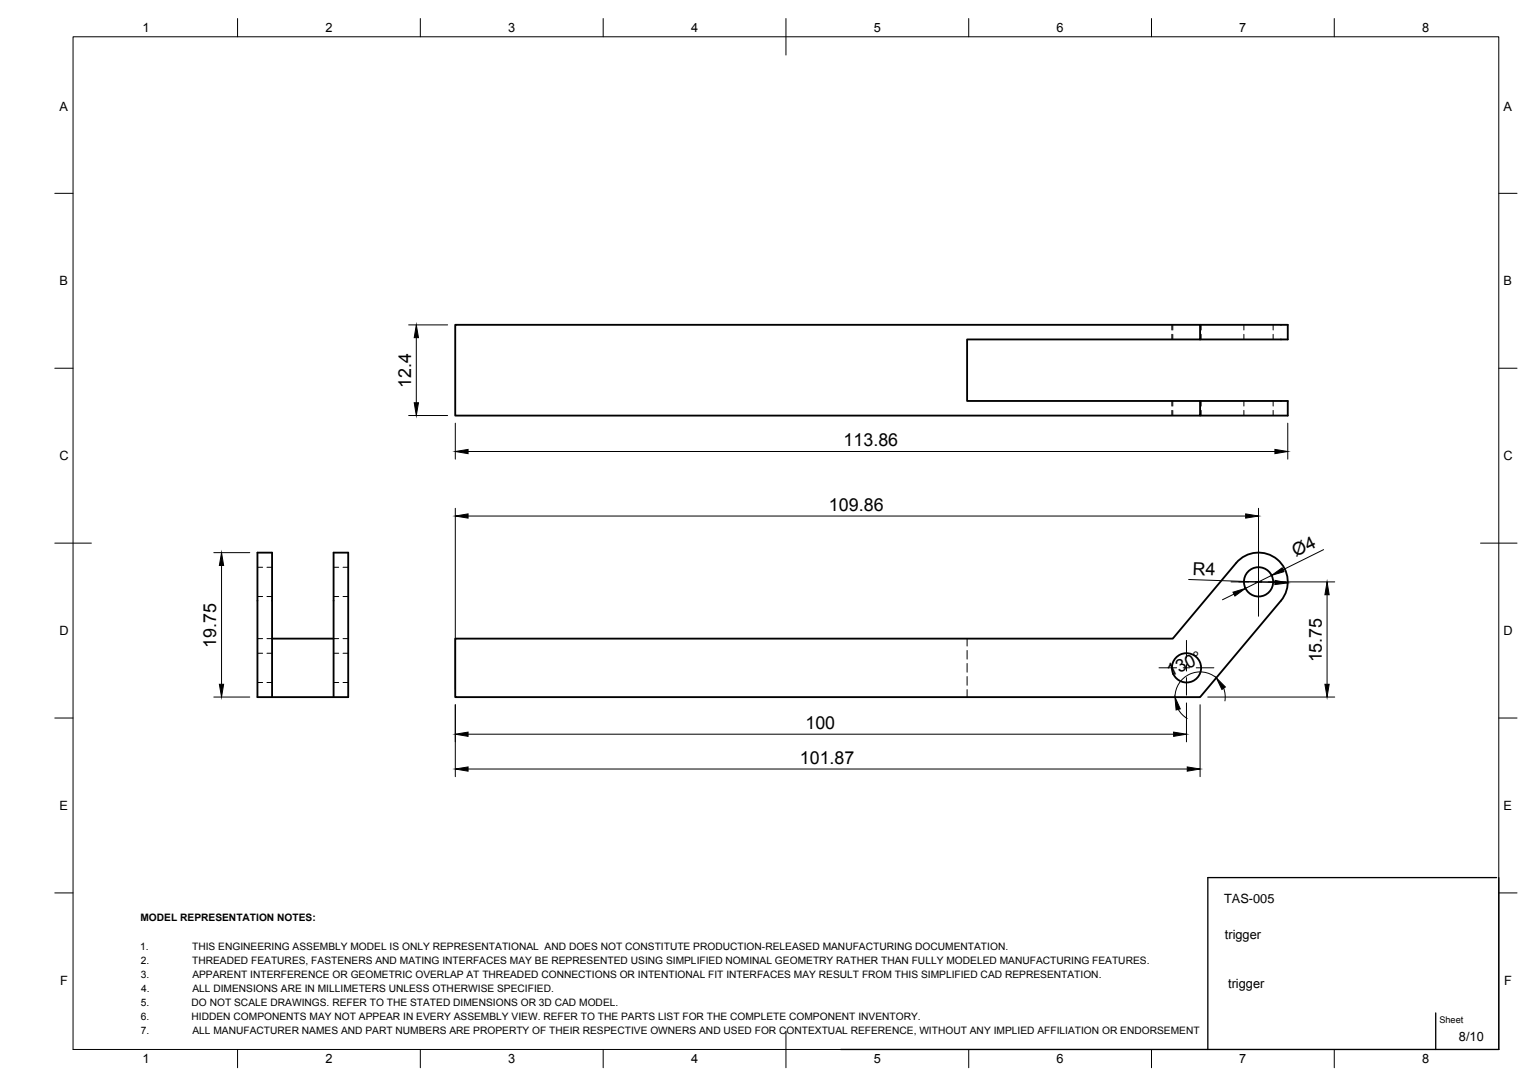
ISO-10303-21;
HEADER;
/* Generated by software containing ST-Developer
 * from STEP Tools, Inc. (www.steptools.com) 
 */

FILE_DESCRIPTION(
/* description */ ('STEP AP214'),
/* implementation_level */ '2;1');

FILE_NAME(
/* name */ 'trigger.step',
/* time_stamp */ '2026-11-04T19:54:22-08:00',
/* author */ (''),
/* organization */ (''),
/* preprocessor_version */ 'ST-DEVELOPER v20.2',
/* originating_system */ 'Autodesk Translation Framework v15.17.0.0',
/* authorisation */ '');

FILE_SCHEMA (('AUTOMOTIVE_DESIGN { 1 0 10303 214 3 1 1 }'));
ENDSEC;

DATA;
#10=MECHANICAL_DESIGN_GEOMETRIC_PRESENTATION_REPRESENTATION('',(#244),#14084);
#226=SHAPE_REPRESENTATION_RELATIONSHIP('SRR','None',#14125,#235);
#235=ADVANCED_BREP_SHAPE_REPRESENTATION('',(#253),#14080);
#244=STYLED_ITEM('',(#14175),#253);
#253=MANIFOLD_SOLID_BREP('Body1',#3470);
#273=FACE_BOUND('',#716,.T.);
#274=FACE_BOUND('',#717,.T.);
#275=FACE_BOUND('',#719,.T.);
#276=FACE_BOUND('',#720,.T.);
#277=FACE_BOUND('',#725,.T.);
#278=FACE_BOUND('',#726,.T.);
#279=FACE_BOUND('',#728,.T.);
#280=FACE_BOUND('',#729,.T.);
#338=PLANE('',#3779);
#339=PLANE('',#3780);
#340=PLANE('',#3781);
#341=PLANE('',#3782);
#342=PLANE('',#3783);
#343=PLANE('',#3784);
#344=PLANE('',#3785);
#345=PLANE('',#3786);
#346=PLANE('',#3787);
#347=PLANE('',#3788);
#348=PLANE('',#3789);
#349=PLANE('',#3791);
#499=FACE_OUTER_BOUND('',#705,.T.);
#500=FACE_OUTER_BOUND('',#706,.T.);
#501=FACE_OUTER_BOUND('',#707,.T.);
#502=FACE_OUTER_BOUND('',#708,.T.);
#503=FACE_OUTER_BOUND('',#709,.T.);
#504=FACE_OUTER_BOUND('',#710,.T.);
#505=FACE_OUTER_BOUND('',#711,.T.);
#506=FACE_OUTER_BOUND('',#712,.T.);
#507=FACE_OUTER_BOUND('',#713,.T.);
#508=FACE_OUTER_BOUND('',#714,.T.);
#509=FACE_OUTER_BOUND('',#715,.T.);
#510=FACE_OUTER_BOUND('',#718,.T.);
#511=FACE_OUTER_BOUND('',#721,.T.);
#512=FACE_OUTER_BOUND('',#722,.T.);
#513=FACE_OUTER_BOUND('',#723,.T.);
#514=FACE_OUTER_BOUND('',#724,.T.);
#515=FACE_OUTER_BOUND('',#727,.T.);
#516=FACE_OUTER_BOUND('',#730,.T.);
#705=EDGE_LOOP('',(#2935,#2936,#2937,#2938));
#706=EDGE_LOOP('',(#2939,#2940,#2941,#2942));
#707=EDGE_LOOP('',(#2943,#2944,#2945,#2946));
#708=EDGE_LOOP('',(#2947,#2948,#2949,#2950));
#709=EDGE_LOOP('',(#2951,#2952,#2953,#2954));
#710=EDGE_LOOP('',(#2955,#2956,#2957,#2958,#2959,#2960,#2961,#2962));
#711=EDGE_LOOP('',(#2963,#2964,#2965,#2966));
#712=EDGE_LOOP('',(#2967,#2968,#2969,#2970,#2971,#2972,#2973,#2974));
#713=EDGE_LOOP('',(#2975,#2976,#2977,#2978));
#714=EDGE_LOOP('',(#2979,#2980,#2981,#2982));
#715=EDGE_LOOP('',(#2983,#2984,#2985,#2986,#2987,#2988));
#716=EDGE_LOOP('',(#2989));
#717=EDGE_LOOP('',(#2990));
#718=EDGE_LOOP('',(#2991,#2992,#2993,#2994,#2995,#2996));
#719=EDGE_LOOP('',(#2997));
#720=EDGE_LOOP('',(#2998));
#721=EDGE_LOOP('',(#2999,#3000,#3001,#3002));
#722=EDGE_LOOP('',(#3003,#3004,#3005,#3006));
#723=EDGE_LOOP('',(#3007,#3008,#3009,#3010));
#724=EDGE_LOOP('',(#3011,#3012,#3013,#3014,#3015,#3016));
#725=EDGE_LOOP('',(#3017));
#726=EDGE_LOOP('',(#3018));
#727=EDGE_LOOP('',(#3019,#3020,#3021,#3022,#3023,#3024));
#728=EDGE_LOOP('',(#3025));
#729=EDGE_LOOP('',(#3026));
#730=EDGE_LOOP('',(#3027,#3028,#3029,#3030));
#979=LINE('',#9274,#1236);
#980=LINE('',#9280,#1237);
#981=LINE('',#9286,#1238);
#982=LINE('',#9292,#1239);
#983=LINE('',#9299,#1240);
#984=LINE('',#9302,#1241);
#985=LINE('',#9306,#1242);
#986=LINE('',#9308,#1243);
#987=LINE('',#9310,#1244);
#988=LINE('',#9312,#1245);
#989=LINE('',#9314,#1246);
#990=LINE('',#9316,#1247);
#991=LINE('',#9318,#1248);
#992=LINE('',#9319,#1249);
#993=LINE('',#9322,#1250);
#994=LINE('',#9324,#1251);
#995=LINE('',#9325,#1252);
#996=LINE('',#9328,#1253);
#997=LINE('',#9330,#1254);
#998=LINE('',#9332,#1255);
#999=LINE('',#9334,#1256);
#1000=LINE('',#9336,#1257);
#1001=LINE('',#9338,#1258);
#1002=LINE('',#9339,#1259);
#1003=LINE('',#9341,#1260);
#1004=LINE('',#9342,#1261);
#1005=LINE('',#9344,#1262);
#1006=LINE('',#9345,#1263);
#1007=LINE('',#9348,#1264);
#1008=LINE('',#9350,#1265);
#1009=LINE('',#9353,#1266);
#1010=LINE('',#9355,#1267);
#1011=LINE('',#9356,#1268);
#1012=LINE('',#9359,#1269);
#1013=LINE('',#9361,#1270);
#1014=LINE('',#9362,#1271);
#1236=VECTOR('',#4454,2.);
#1237=VECTOR('',#4461,2.);
#1238=VECTOR('',#4468,2.);
#1239=VECTOR('',#4475,2.);
#1240=VECTOR('',#4482,1000.);
#1241=VECTOR('',#4485,1000.);
#1242=VECTOR('',#4488,1000.);
#1243=VECTOR('',#4489,1000.);
#1244=VECTOR('',#4490,1000.);
#1245=VECTOR('',#4491,1000.);
#1246=VECTOR('',#4492,1000.);
#1247=VECTOR('',#4493,1000.);
#1248=VECTOR('',#4494,1000.);
#1249=VECTOR('',#4495,1000.);
#1250=VECTOR('',#4498,1000.);
#1251=VECTOR('',#4499,1000.);
#1252=VECTOR('',#4500,1000.);
#1253=VECTOR('',#4503,1000.);
#1254=VECTOR('',#4504,1000.);
#1255=VECTOR('',#4505,1000.);
#1256=VECTOR('',#4506,1000.);
#1257=VECTOR('',#4507,1000.);
#1258=VECTOR('',#4508,1000.);
#1259=VECTOR('',#4509,1000.);
#1260=VECTOR('',#4512,1000.);
#1261=VECTOR('',#4513,1000.);
#1262=VECTOR('',#4516,1000.);
#1263=VECTOR('',#4517,1000.);
#1264=VECTOR('',#4522,1000.);
#1265=VECTOR('',#4525,1000.);
#1266=VECTOR('',#4528,1000.);
#1267=VECTOR('',#4529,1000.);
#1268=VECTOR('',#4530,1000.);
#1269=VECTOR('',#4533,1000.);
#1270=VECTOR('',#4534,1000.);
#1271=VECTOR('',#4535,1000.);
#1338=CIRCLE('',#3765,2.);
#1339=CIRCLE('',#3766,2.);
#1340=CIRCLE('',#3768,2.);
#1341=CIRCLE('',#3769,2.);
#1342=CIRCLE('',#3771,2.);
#1343=CIRCLE('',#3772,2.);
#1344=CIRCLE('',#3774,2.);
#1345=CIRCLE('',#3775,2.);
#1346=CIRCLE('',#3777,4.);
#1347=CIRCLE('',#3778,4.);
#1348=CIRCLE('',#3790,4.);
#1349=CIRCLE('',#3792,4.);
#1622=VERTEX_POINT('',#9271);
#1623=VERTEX_POINT('',#9273);
#1624=VERTEX_POINT('',#9277);
#1625=VERTEX_POINT('',#9279);
#1626=VERTEX_POINT('',#9283);
#1627=VERTEX_POINT('',#9285);
#1628=VERTEX_POINT('',#9289);
#1629=VERTEX_POINT('',#9291);
#1630=VERTEX_POINT('',#9295);
#1631=VERTEX_POINT('',#9296);
#1632=VERTEX_POINT('',#9298);
#1633=VERTEX_POINT('',#9300);
#1634=VERTEX_POINT('',#9304);
#1635=VERTEX_POINT('',#9305);
#1636=VERTEX_POINT('',#9307);
#1637=VERTEX_POINT('',#9309);
#1638=VERTEX_POINT('',#9311);
#1639=VERTEX_POINT('',#9313);
#1640=VERTEX_POINT('',#9315);
#1641=VERTEX_POINT('',#9317);
#1642=VERTEX_POINT('',#9321);
#1643=VERTEX_POINT('',#9323);
#1644=VERTEX_POINT('',#9327);
#1645=VERTEX_POINT('',#9329);
#1646=VERTEX_POINT('',#9331);
#1647=VERTEX_POINT('',#9333);
#1648=VERTEX_POINT('',#9335);
#1649=VERTEX_POINT('',#9337);
#1650=VERTEX_POINT('',#9352);
#1651=VERTEX_POINT('',#9354);
#1652=VERTEX_POINT('',#9358);
#1653=VERTEX_POINT('',#9360);
#2071=EDGE_CURVE('',#1622,#1622,#1338,.T.);
#2072=EDGE_CURVE('',#1622,#1623,#979,.T.);
#2073=EDGE_CURVE('',#1623,#1623,#1339,.T.);
#2074=EDGE_CURVE('',#1624,#1624,#1340,.T.);
#2075=EDGE_CURVE('',#1624,#1625,#980,.T.);
#2076=EDGE_CURVE('',#1625,#1625,#1341,.T.);
#2077=EDGE_CURVE('',#1626,#1626,#1342,.T.);
#2078=EDGE_CURVE('',#1626,#1627,#981,.T.);
#2079=EDGE_CURVE('',#1627,#1627,#1343,.T.);
#2080=EDGE_CURVE('',#1628,#1628,#1344,.T.);
#2081=EDGE_CURVE('',#1628,#1629,#982,.T.);
#2082=EDGE_CURVE('',#1629,#1629,#1345,.T.);
#2083=EDGE_CURVE('',#1630,#1631,#1346,.T.);
#2084=EDGE_CURVE('',#1632,#1630,#983,.T.);
#2085=EDGE_CURVE('',#1633,#1632,#1347,.T.);
#2086=EDGE_CURVE('',#1631,#1633,#984,.T.);
#2087=EDGE_CURVE('',#1634,#1635,#985,.T.);
#2088=EDGE_CURVE('',#1636,#1635,#986,.T.);
#2089=EDGE_CURVE('',#1637,#1636,#987,.T.);
#2090=EDGE_CURVE('',#1638,#1637,#988,.T.);
#2091=EDGE_CURVE('',#1638,#1639,#989,.T.);
#2092=EDGE_CURVE('',#1640,#1639,#990,.T.);
#2093=EDGE_CURVE('',#1641,#1640,#991,.T.);
#2094=EDGE_CURVE('',#1641,#1634,#992,.T.);
#2095=EDGE_CURVE('',#1642,#1639,#993,.T.);
#2096=EDGE_CURVE('',#1643,#1642,#994,.T.);
#2097=EDGE_CURVE('',#1643,#1640,#995,.T.);
#2098=EDGE_CURVE('',#1644,#1643,#996,.T.);
#2099=EDGE_CURVE('',#1645,#1642,#997,.T.);
#2100=EDGE_CURVE('',#1645,#1646,#998,.T.);
#2101=EDGE_CURVE('',#1646,#1647,#999,.T.);
#2102=EDGE_CURVE('',#1647,#1648,#1000,.T.);
#2103=EDGE_CURVE('',#1649,#1648,#1001,.T.);
#2104=EDGE_CURVE('',#1644,#1649,#1002,.T.);
#2105=EDGE_CURVE('',#1632,#1649,#1003,.T.);
#2106=EDGE_CURVE('',#1630,#1644,#1004,.T.);
#2107=EDGE_CURVE('',#1631,#1641,#1005,.T.);
#2108=EDGE_CURVE('',#1633,#1634,#1006,.T.);
#2109=EDGE_CURVE('',#1635,#1648,#1007,.T.);
#2110=EDGE_CURVE('',#1636,#1647,#1008,.T.);
#2111=EDGE_CURVE('',#1650,#1646,#1009,.T.);
#2112=EDGE_CURVE('',#1651,#1645,#1010,.T.);
#2113=EDGE_CURVE('',#1650,#1651,#1011,.T.);
#2114=EDGE_CURVE('',#1652,#1638,#1012,.T.);
#2115=EDGE_CURVE('',#1653,#1637,#1013,.T.);
#2116=EDGE_CURVE('',#1652,#1653,#1014,.T.);
#2117=EDGE_CURVE('',#1651,#1652,#1348,.T.);
#2118=EDGE_CURVE('',#1653,#1650,#1349,.T.);
#2935=ORIENTED_EDGE('',*,*,#2071,.T.);
#2936=ORIENTED_EDGE('',*,*,#2072,.T.);
#2937=ORIENTED_EDGE('',*,*,#2073,.T.);
#2938=ORIENTED_EDGE('',*,*,#2072,.F.);
#2939=ORIENTED_EDGE('',*,*,#2074,.F.);
#2940=ORIENTED_EDGE('',*,*,#2075,.T.);
#2941=ORIENTED_EDGE('',*,*,#2076,.T.);
#2942=ORIENTED_EDGE('',*,*,#2075,.F.);
#2943=ORIENTED_EDGE('',*,*,#2077,.T.);
#2944=ORIENTED_EDGE('',*,*,#2078,.T.);
#2945=ORIENTED_EDGE('',*,*,#2079,.T.);
#2946=ORIENTED_EDGE('',*,*,#2078,.F.);
#2947=ORIENTED_EDGE('',*,*,#2080,.F.);
#2948=ORIENTED_EDGE('',*,*,#2081,.T.);
#2949=ORIENTED_EDGE('',*,*,#2082,.T.);
#2950=ORIENTED_EDGE('',*,*,#2081,.F.);
#2951=ORIENTED_EDGE('',*,*,#2083,.F.);
#2952=ORIENTED_EDGE('',*,*,#2084,.F.);
#2953=ORIENTED_EDGE('',*,*,#2085,.F.);
#2954=ORIENTED_EDGE('',*,*,#2086,.F.);
#2955=ORIENTED_EDGE('',*,*,#2087,.T.);
#2956=ORIENTED_EDGE('',*,*,#2088,.F.);
#2957=ORIENTED_EDGE('',*,*,#2089,.F.);
#2958=ORIENTED_EDGE('',*,*,#2090,.F.);
#2959=ORIENTED_EDGE('',*,*,#2091,.T.);
#2960=ORIENTED_EDGE('',*,*,#2092,.F.);
#2961=ORIENTED_EDGE('',*,*,#2093,.F.);
#2962=ORIENTED_EDGE('',*,*,#2094,.T.);
#2963=ORIENTED_EDGE('',*,*,#2092,.T.);
#2964=ORIENTED_EDGE('',*,*,#2095,.F.);
#2965=ORIENTED_EDGE('',*,*,#2096,.F.);
#2966=ORIENTED_EDGE('',*,*,#2097,.T.);
#2967=ORIENTED_EDGE('',*,*,#2098,.T.);
#2968=ORIENTED_EDGE('',*,*,#2096,.T.);
#2969=ORIENTED_EDGE('',*,*,#2099,.F.);
#2970=ORIENTED_EDGE('',*,*,#2100,.T.);
#2971=ORIENTED_EDGE('',*,*,#2101,.T.);
#2972=ORIENTED_EDGE('',*,*,#2102,.T.);
#2973=ORIENTED_EDGE('',*,*,#2103,.F.);
#2974=ORIENTED_EDGE('',*,*,#2104,.F.);
#2975=ORIENTED_EDGE('',*,*,#2105,.F.);
#2976=ORIENTED_EDGE('',*,*,#2084,.T.);
#2977=ORIENTED_EDGE('',*,*,#2106,.T.);
#2978=ORIENTED_EDGE('',*,*,#2104,.T.);
#2979=ORIENTED_EDGE('',*,*,#2107,.F.);
#2980=ORIENTED_EDGE('',*,*,#2086,.T.);
#2981=ORIENTED_EDGE('',*,*,#2108,.T.);
#2982=ORIENTED_EDGE('',*,*,#2094,.F.);
#2983=ORIENTED_EDGE('',*,*,#2097,.F.);
#2984=ORIENTED_EDGE('',*,*,#2098,.F.);
#2985=ORIENTED_EDGE('',*,*,#2106,.F.);
#2986=ORIENTED_EDGE('',*,*,#2083,.T.);
#2987=ORIENTED_EDGE('',*,*,#2107,.T.);
#2988=ORIENTED_EDGE('',*,*,#2093,.T.);
#2989=ORIENTED_EDGE('',*,*,#2073,.F.);
#2990=ORIENTED_EDGE('',*,*,#2079,.F.);
#2991=ORIENTED_EDGE('',*,*,#2109,.F.);
#2992=ORIENTED_EDGE('',*,*,#2087,.F.);
#2993=ORIENTED_EDGE('',*,*,#2108,.F.);
#2994=ORIENTED_EDGE('',*,*,#2085,.T.);
#2995=ORIENTED_EDGE('',*,*,#2105,.T.);
#2996=ORIENTED_EDGE('',*,*,#2103,.T.);
#2997=ORIENTED_EDGE('',*,*,#2071,.F.);
#2998=ORIENTED_EDGE('',*,*,#2077,.F.);
#2999=ORIENTED_EDGE('',*,*,#2088,.T.);
#3000=ORIENTED_EDGE('',*,*,#2109,.T.);
#3001=ORIENTED_EDGE('',*,*,#2102,.F.);
#3002=ORIENTED_EDGE('',*,*,#2110,.F.);
#3003=ORIENTED_EDGE('',*,*,#2111,.T.);
#3004=ORIENTED_EDGE('',*,*,#2100,.F.);
#3005=ORIENTED_EDGE('',*,*,#2112,.F.);
#3006=ORIENTED_EDGE('',*,*,#2113,.F.);
#3007=ORIENTED_EDGE('',*,*,#2114,.T.);
#3008=ORIENTED_EDGE('',*,*,#2090,.T.);
#3009=ORIENTED_EDGE('',*,*,#2115,.F.);
#3010=ORIENTED_EDGE('',*,*,#2116,.F.);
#3011=ORIENTED_EDGE('',*,*,#2112,.T.);
#3012=ORIENTED_EDGE('',*,*,#2099,.T.);
#3013=ORIENTED_EDGE('',*,*,#2095,.T.);
#3014=ORIENTED_EDGE('',*,*,#2091,.F.);
#3015=ORIENTED_EDGE('',*,*,#2114,.F.);
#3016=ORIENTED_EDGE('',*,*,#2117,.F.);
#3017=ORIENTED_EDGE('',*,*,#2074,.T.);
#3018=ORIENTED_EDGE('',*,*,#2080,.T.);
#3019=ORIENTED_EDGE('',*,*,#2089,.T.);
#3020=ORIENTED_EDGE('',*,*,#2110,.T.);
#3021=ORIENTED_EDGE('',*,*,#2101,.F.);
#3022=ORIENTED_EDGE('',*,*,#2111,.F.);
#3023=ORIENTED_EDGE('',*,*,#2118,.F.);
#3024=ORIENTED_EDGE('',*,*,#2115,.T.);
#3025=ORIENTED_EDGE('',*,*,#2076,.F.);
#3026=ORIENTED_EDGE('',*,*,#2082,.F.);
#3027=ORIENTED_EDGE('',*,*,#2116,.T.);
#3028=ORIENTED_EDGE('',*,*,#2118,.T.);
#3029=ORIENTED_EDGE('',*,*,#2113,.T.);
#3030=ORIENTED_EDGE('',*,*,#2117,.T.);
#3264=CYLINDRICAL_SURFACE('',#3764,2.);
#3265=CYLINDRICAL_SURFACE('',#3767,2.);
#3266=CYLINDRICAL_SURFACE('',#3770,2.);
#3267=CYLINDRICAL_SURFACE('',#3773,2.);
#3268=CYLINDRICAL_SURFACE('',#3776,4.);
#3269=CYLINDRICAL_SURFACE('',#3793,4.);
#3409=ADVANCED_FACE('',(#499),#3264,.F.);
#3410=ADVANCED_FACE('',(#500),#3265,.F.);
#3411=ADVANCED_FACE('',(#501),#3266,.F.);
#3412=ADVANCED_FACE('',(#502),#3267,.F.);
#3413=ADVANCED_FACE('',(#503),#3268,.T.);
#3414=ADVANCED_FACE('',(#504),#338,.F.);
#3415=ADVANCED_FACE('',(#505),#339,.T.);
#3416=ADVANCED_FACE('',(#506),#340,.T.);
#3417=ADVANCED_FACE('',(#507),#341,.T.);
#3418=ADVANCED_FACE('',(#508),#342,.F.);
#3419=ADVANCED_FACE('',(#509,#273,#274),#343,.F.);
#3420=ADVANCED_FACE('',(#510,#275,#276),#344,.T.);
#3421=ADVANCED_FACE('',(#511),#345,.T.);
#3422=ADVANCED_FACE('',(#512),#346,.T.);
#3423=ADVANCED_FACE('',(#513),#347,.F.);
#3424=ADVANCED_FACE('',(#514,#277,#278),#348,.F.);
#3425=ADVANCED_FACE('',(#515,#279,#280),#349,.T.);
#3426=ADVANCED_FACE('',(#516),#3269,.T.);
#3470=CLOSED_SHELL('',(#3409,#3410,#3411,#3412,#3413,#3414,#3415,#3416,
#3417,#3418,#3419,#3420,#3421,#3422,#3423,#3424,#3425,#3426));
#3763=AXIS2_PLACEMENT_3D('',#9269,#4448,#4449);
#3764=AXIS2_PLACEMENT_3D('',#9270,#4450,#4451);
#3765=AXIS2_PLACEMENT_3D('',#9272,#4452,#4453);
#3766=AXIS2_PLACEMENT_3D('',#9275,#4455,#4456);
#3767=AXIS2_PLACEMENT_3D('',#9276,#4457,#4458);
#3768=AXIS2_PLACEMENT_3D('',#9278,#4459,#4460);
#3769=AXIS2_PLACEMENT_3D('',#9281,#4462,#4463);
#3770=AXIS2_PLACEMENT_3D('',#9282,#4464,#4465);
#3771=AXIS2_PLACEMENT_3D('',#9284,#4466,#4467);
#3772=AXIS2_PLACEMENT_3D('',#9287,#4469,#4470);
#3773=AXIS2_PLACEMENT_3D('',#9288,#4471,#4472);
#3774=AXIS2_PLACEMENT_3D('',#9290,#4473,#4474);
#3775=AXIS2_PLACEMENT_3D('',#9293,#4476,#4477);
#3776=AXIS2_PLACEMENT_3D('',#9294,#4478,#4479);
#3777=AXIS2_PLACEMENT_3D('',#9297,#4480,#4481);
#3778=AXIS2_PLACEMENT_3D('',#9301,#4483,#4484);
#3779=AXIS2_PLACEMENT_3D('',#9303,#4486,#4487);
#3780=AXIS2_PLACEMENT_3D('',#9320,#4496,#4497);
#3781=AXIS2_PLACEMENT_3D('',#9326,#4501,#4502);
#3782=AXIS2_PLACEMENT_3D('',#9340,#4510,#4511);
#3783=AXIS2_PLACEMENT_3D('',#9343,#4514,#4515);
#3784=AXIS2_PLACEMENT_3D('',#9346,#4518,#4519);
#3785=AXIS2_PLACEMENT_3D('',#9347,#4520,#4521);
#3786=AXIS2_PLACEMENT_3D('',#9349,#4523,#4524);
#3787=AXIS2_PLACEMENT_3D('',#9351,#4526,#4527);
#3788=AXIS2_PLACEMENT_3D('',#9357,#4531,#4532);
#3789=AXIS2_PLACEMENT_3D('',#9363,#4536,#4537);
#3790=AXIS2_PLACEMENT_3D('',#9364,#4538,#4539);
#3791=AXIS2_PLACEMENT_3D('',#9365,#4540,#4541);
#3792=AXIS2_PLACEMENT_3D('',#9366,#4542,#4543);
#3793=AXIS2_PLACEMENT_3D('',#9367,#4544,#4545);
#4448=DIRECTION('axis',(0.,0.,1.));
#4449=DIRECTION('refdir',(1.,0.,0.));
#4450=DIRECTION('center_axis',(0.,0.,1.));
#4451=DIRECTION('ref_axis',(1.,0.,0.));
#4452=DIRECTION('center_axis',(0.,0.,-1.));
#4453=DIRECTION('ref_axis',(-1.,0.,0.));
#4454=DIRECTION('',(0.,0.,1.));
#4455=DIRECTION('center_axis',(0.,0.,1.));
#4456=DIRECTION('ref_axis',(1.,0.,0.));
#4457=DIRECTION('center_axis',(0.,0.,1.));
#4458=DIRECTION('ref_axis',(1.,0.,0.));
#4459=DIRECTION('center_axis',(0.,0.,1.));
#4460=DIRECTION('ref_axis',(1.,0.,0.));
#4461=DIRECTION('',(0.,0.,1.));
#4462=DIRECTION('center_axis',(0.,0.,1.));
#4463=DIRECTION('ref_axis',(1.,0.,0.));
#4464=DIRECTION('center_axis',(0.,0.,1.));
#4465=DIRECTION('ref_axis',(1.,0.,0.));
#4466=DIRECTION('center_axis',(0.,0.,-1.));
#4467=DIRECTION('ref_axis',(-1.,0.,0.));
#4468=DIRECTION('',(0.,0.,1.));
#4469=DIRECTION('center_axis',(0.,0.,1.));
#4470=DIRECTION('ref_axis',(1.,0.,0.));
#4471=DIRECTION('center_axis',(0.,0.,1.));
#4472=DIRECTION('ref_axis',(1.,0.,0.));
#4473=DIRECTION('center_axis',(0.,0.,1.));
#4474=DIRECTION('ref_axis',(1.,0.,0.));
#4475=DIRECTION('',(0.,0.,1.));
#4476=DIRECTION('center_axis',(0.,0.,1.));
#4477=DIRECTION('ref_axis',(1.,0.,0.));
#4478=DIRECTION('center_axis',(0.,0.,-1.));
#4479=DIRECTION('ref_axis',(-1.,0.,0.));
#4480=DIRECTION('center_axis',(0.,0.,1.));
#4481=DIRECTION('ref_axis',(-1.,0.,0.));
#4482=DIRECTION('',(0.,0.,1.));
#4483=DIRECTION('center_axis',(0.,0.,-1.));
#4484=DIRECTION('ref_axis',(-1.,0.,0.));
#4485=DIRECTION('',(0.,0.,-1.));
#4486=DIRECTION('center_axis',(0.415719046892318,0.909493086312888,0.));
#4487=DIRECTION('ref_axis',(-0.909493086312888,0.415719046892318,0.));
#4488=DIRECTION('',(0.909493086312888,-0.415719046892318,0.));
#4489=DIRECTION('',(0.,0.,1.));
#4490=DIRECTION('',(0.909493086312888,-0.415719046892318,0.));
#4491=DIRECTION('',(0.,0.,1.));
#4492=DIRECTION('',(0.909493086312888,-0.415719046892318,0.));
#4493=DIRECTION('',(0.,0.,-1.));
#4494=DIRECTION('',(0.909493086312888,-0.415719046892318,0.));
#4495=DIRECTION('',(0.,0.,-1.));
#4496=DIRECTION('center_axis',(0.909493086312887,-0.41571904689232,0.));
#4497=DIRECTION('ref_axis',(0.41571904689232,0.909493086312887,0.));
#4498=DIRECTION('',(-0.41571904689232,-0.909493086312887,0.));
#4499=DIRECTION('',(0.,0.,-1.));
#4500=DIRECTION('',(-0.41571904689232,-0.909493086312887,0.));
#4501=DIRECTION('center_axis',(0.415719046892318,0.909493086312888,0.));
#4502=DIRECTION('ref_axis',(-0.909493086312888,0.415719046892318,0.));
#4503=DIRECTION('',(0.909493086312888,-0.415719046892318,0.));
#4504=DIRECTION('',(0.909493086312888,-0.415719046892318,0.));
#4505=DIRECTION('',(0.,0.,1.));
#4506=DIRECTION('',(0.909493086312888,-0.415719046892318,0.));
#4507=DIRECTION('',(0.,0.,1.));
#4508=DIRECTION('',(0.909493086312888,-0.415719046892318,0.));
#4509=DIRECTION('',(0.,0.,-1.));
#4510=DIRECTION('center_axis',(-0.42949307237204,0.903070152748072,0.));
#4511=DIRECTION('ref_axis',(-0.903070152748072,-0.42949307237204,0.));
#4512=DIRECTION('',(0.903070152748072,0.42949307237204,0.));
#4513=DIRECTION('',(0.903070152748072,0.42949307237204,0.));
#4514=DIRECTION('center_axis',(-0.42949307237204,0.903070152748072,0.));
#4515=DIRECTION('ref_axis',(-0.903070152748072,-0.42949307237204,0.));
#4516=DIRECTION('',(0.903070152748072,0.42949307237204,0.));
#4517=DIRECTION('',(0.903070152748072,0.42949307237204,0.));
#4518=DIRECTION('center_axis',(0.,0.,-1.));
#4519=DIRECTION('ref_axis',(-1.,0.,0.));
#4520=DIRECTION('center_axis',(0.,0.,-1.));
#4521=DIRECTION('ref_axis',(-1.,0.,0.));
#4522=DIRECTION('',(0.415719046892314,0.90949308631289,0.));
#4523=DIRECTION('center_axis',(-0.90949308631289,0.415719046892314,0.));
#4524=DIRECTION('ref_axis',(-0.415719046892314,-0.90949308631289,0.));
#4525=DIRECTION('',(0.415719046892314,0.90949308631289,0.));
#4526=DIRECTION('center_axis',(-0.42949307237204,0.903070152748072,0.));
#4527=DIRECTION('ref_axis',(-0.903070152748072,-0.42949307237204,0.));
#4528=DIRECTION('',(0.903070152748072,0.42949307237204,0.));
#4529=DIRECTION('',(0.903070152748072,0.42949307237204,0.));
#4530=DIRECTION('',(0.,0.,-1.));
#4531=DIRECTION('center_axis',(-0.42949307237204,0.903070152748072,0.));
#4532=DIRECTION('ref_axis',(-0.903070152748072,-0.42949307237204,0.));
#4533=DIRECTION('',(0.903070152748072,0.42949307237204,0.));
#4534=DIRECTION('',(0.903070152748072,0.42949307237204,0.));
#4535=DIRECTION('',(0.,0.,1.));
#4536=DIRECTION('center_axis',(0.,0.,1.));
#4537=DIRECTION('ref_axis',(-1.,0.,0.));
#4538=DIRECTION('center_axis',(0.,0.,1.));
#4539=DIRECTION('ref_axis',(-1.,0.,0.));
#4540=DIRECTION('center_axis',(0.,0.,1.));
#4541=DIRECTION('ref_axis',(-1.,0.,0.));
#4542=DIRECTION('center_axis',(0.,0.,-1.));
#4543=DIRECTION('ref_axis',(-1.,0.,0.));
#4544=DIRECTION('center_axis',(0.,0.,-1.));
#4545=DIRECTION('ref_axis',(-0.903070152748072,-0.429493072372039,0.));
#9269=CARTESIAN_POINT('',(0.,0.,0.));
#9270=CARTESIAN_POINT('Origin',(32.,329.539392014169,6.2));
#9271=CARTESIAN_POINT('',(30.,329.539392014169,4.2));
#9272=CARTESIAN_POINT('Origin',(32.,329.539392014169,4.2));
#9273=CARTESIAN_POINT('',(30.,329.539392014169,6.2));
#9274=CARTESIAN_POINT('',(30.,329.539392014169,6.2));
#9275=CARTESIAN_POINT('Origin',(32.,329.539392014169,6.2));
#9276=CARTESIAN_POINT('Origin',(32.,329.539392014169,6.2));
#9277=CARTESIAN_POINT('',(30.,329.539392014169,-6.2));
#9278=CARTESIAN_POINT('Origin',(32.,329.539392014169,-6.2));
#9279=CARTESIAN_POINT('',(30.,329.539392014169,-4.2));
#9280=CARTESIAN_POINT('',(30.,329.539392014169,6.2));
#9281=CARTESIAN_POINT('Origin',(32.,329.539392014169,-4.2));
#9282=CARTESIAN_POINT('Origin',(18.1535684584702,322.954137916175,6.2));
#9283=CARTESIAN_POINT('',(16.1535684584702,322.954137916175,4.2));
#9284=CARTESIAN_POINT('Origin',(18.1535684584702,322.954137916175,4.2));
#9285=CARTESIAN_POINT('',(16.1535684584702,322.954137916175,6.2));
#9286=CARTESIAN_POINT('',(16.1535684584702,322.954137916175,6.2));
#9287=CARTESIAN_POINT('Origin',(18.1535684584702,322.954137916175,6.2));
#9288=CARTESIAN_POINT('Origin',(18.1535684584702,322.954137916175,6.2));
#9289=CARTESIAN_POINT('',(16.1535684584702,322.954137916175,-6.2));
#9290=CARTESIAN_POINT('Origin',(18.1535684584702,322.954137916175,-6.2));
#9291=CARTESIAN_POINT('',(16.1535684584702,322.954137916175,-4.2));
#9292=CARTESIAN_POINT('',(16.1535684584702,322.954137916175,6.2));
#9293=CARTESIAN_POINT('Origin',(18.1535684584702,322.954137916175,-4.2));
#9294=CARTESIAN_POINT('Origin',(18.1535684584702,322.954137916175,6.2));
#9295=CARTESIAN_POINT('',(16.4355961689821,326.566418527167,6.2));
#9296=CARTESIAN_POINT('',(19.8715407479584,319.341857305183,6.2));
#9297=CARTESIAN_POINT('Origin',(18.1535684584702,322.954137916175,6.2));
#9298=CARTESIAN_POINT('',(16.4355961689821,326.566418527167,4.2));
#9299=CARTESIAN_POINT('',(16.4355961689821,326.566418527167,6.2));
#9300=CARTESIAN_POINT('',(19.8715407479584,319.341857305183,4.2));
#9301=CARTESIAN_POINT('Origin',(18.1535684584702,322.954137916175,4.2));
#9302=CARTESIAN_POINT('',(19.8715407479584,319.341857305183,4.2));
#9303=CARTESIAN_POINT('Origin',(30.3371238124307,325.901419668918,6.2));
#9304=CARTESIAN_POINT('',(32.0335381771776,325.126007768091,4.2));
#9305=CARTESIAN_POINT('',(57.6219164018174,313.429848262148,4.2));
#9306=CARTESIAN_POINT('',(30.3371238124307,325.901419668918,4.2));
#9307=CARTESIAN_POINT('',(57.6219164018174,313.429848262148,-4.20000000000002));
#9308=CARTESIAN_POINT('',(57.6219164018174,313.429848262148,-80.4294540302737));
#9309=CARTESIAN_POINT('',(32.0335381771776,325.126007768091,-4.2));
#9310=CARTESIAN_POINT('',(30.3371238124307,325.901419668918,-4.2));
#9311=CARTESIAN_POINT('',(32.0335381771776,325.126007768091,-6.2));
#9312=CARTESIAN_POINT('',(32.0335381771776,325.126007768091,-6.2));
#9313=CARTESIAN_POINT('',(121.28643244372,284.329514979686,-6.2));
#9314=CARTESIAN_POINT('',(30.3371238124307,325.901419668918,-6.2));
#9315=CARTESIAN_POINT('',(121.28643244372,284.329514979686,6.2));
#9316=CARTESIAN_POINT('',(121.28643244372,284.329514979686,6.2));
#9317=CARTESIAN_POINT('',(32.0335381771776,325.126007768091,6.2));
#9318=CARTESIAN_POINT('',(30.3371238124307,325.901419668918,6.2));
#9319=CARTESIAN_POINT('',(32.0335381771776,325.126007768091,6.2));
#9320=CARTESIAN_POINT('Origin',(124.612184818858,291.605459670189,6.2));
#9321=CARTESIAN_POINT('',(124.612184818858,291.605459670189,-6.2));
#9322=CARTESIAN_POINT('',(124.612184818858,291.605459670189,-6.2));
#9323=CARTESIAN_POINT('',(124.612184818858,291.605459670189,6.2));
#9324=CARTESIAN_POINT('',(124.612184818858,291.605459670189,6.2));
#9325=CARTESIAN_POINT('',(124.612184818858,291.605459670189,6.2));
#9326=CARTESIAN_POINT('Origin',(33.6628761875693,333.177364359421,6.2));
#9327=CARTESIAN_POINT('',(31.9664618228224,333.952776260248,6.2));
#9328=CARTESIAN_POINT('',(33.6628761875693,333.177364359421,6.2));
#9329=CARTESIAN_POINT('',(31.9664618228224,333.952776260248,-6.2));
#9330=CARTESIAN_POINT('',(33.6628761875693,333.177364359421,-6.2));
#9331=CARTESIAN_POINT('',(31.9664618228224,333.952776260248,-4.2));
#9332=CARTESIAN_POINT('',(31.9664618228224,333.952776260248,-6.2));
#9333=CARTESIAN_POINT('',(60.9476687769559,320.705792952651,-4.2));
#9334=CARTESIAN_POINT('',(33.6628761875693,333.177364359421,-4.2));
#9335=CARTESIAN_POINT('',(60.9476687769559,320.705792952651,4.19999999999997));
#9336=CARTESIAN_POINT('',(60.9476687769559,320.705792952651,-80.4294540302737));
#9337=CARTESIAN_POINT('',(31.9664618228224,333.952776260248,4.2));
#9338=CARTESIAN_POINT('',(33.6628761875693,333.177364359421,4.2));
#9339=CARTESIAN_POINT('',(31.9664618228224,333.952776260248,6.2));
#9340=CARTESIAN_POINT('Origin',(12.8233155579898,324.848446237679,6.2));
#9341=CARTESIAN_POINT('',(12.8233155579898,324.848446237679,4.2));
#9342=CARTESIAN_POINT('',(12.8233155579898,324.848446237679,6.2));
#9343=CARTESIAN_POINT('Origin',(16.2592601369661,317.623885015694,6.2));
#9344=CARTESIAN_POINT('',(16.2592601369661,317.623885015694,6.2));
#9345=CARTESIAN_POINT('',(16.2592601369661,317.623885015694,4.2));
#9346=CARTESIAN_POINT('Origin',(0.,0.,6.2));
#9347=CARTESIAN_POINT('Origin',(0.,0.,4.2));
#9348=CARTESIAN_POINT('',(-70.8422565789511,32.3811976450479,4.2));
#9349=CARTESIAN_POINT('Origin',(57.6219164018174,313.429848262148,-80.4294540302737));
#9350=CARTESIAN_POINT('',(57.6219164018174,313.429848262148,-4.2));
#9351=CARTESIAN_POINT('Origin',(12.8233155579898,324.848446237679,-6.2));
#9352=CARTESIAN_POINT('',(16.4355961689821,326.566418527167,-4.2));
#9353=CARTESIAN_POINT('',(12.8233155579898,324.848446237679,-4.2));
#9354=CARTESIAN_POINT('',(16.4355961689821,326.566418527167,-6.2));
#9355=CARTESIAN_POINT('',(12.8233155579898,324.848446237679,-6.2));
#9356=CARTESIAN_POINT('',(16.4355961689821,326.566418527167,-6.2));
#9357=CARTESIAN_POINT('Origin',(16.2592601369661,317.623885015694,-6.2));
#9358=CARTESIAN_POINT('',(19.8715407479584,319.341857305183,-6.2));
#9359=CARTESIAN_POINT('',(16.2592601369661,317.623885015694,-6.2));
#9360=CARTESIAN_POINT('',(19.8715407479584,319.341857305183,-4.2));
#9361=CARTESIAN_POINT('',(16.2592601369661,317.623885015694,-4.2));
#9362=CARTESIAN_POINT('',(19.8715407479584,319.341857305183,-4.2));
#9363=CARTESIAN_POINT('Origin',(0.,0.,-6.2));
#9364=CARTESIAN_POINT('Origin',(18.1535684584702,322.954137916175,-6.2));
#9365=CARTESIAN_POINT('Origin',(0.,0.,-4.2));
#9366=CARTESIAN_POINT('Origin',(18.1535684584702,322.954137916175,-4.2));
#9367=CARTESIAN_POINT('Origin',(18.1535684584702,322.954137916175,-6.2));
#14069=UNCERTAINTY_MEASURE_WITH_UNIT(LENGTH_MEASURE(0.01),#14085,
'DISTANCE_ACCURACY_VALUE',
'Maximum model space distance between geometric entities at asserted c
onnectivities');
#14073=UNCERTAINTY_MEASURE_WITH_UNIT(LENGTH_MEASURE(0.01),#14085,
'DISTANCE_ACCURACY_VALUE',
'Maximum model space distance between geometric entities at asserted c
onnectivities');
#14080=(
GEOMETRIC_REPRESENTATION_CONTEXT(3)
GLOBAL_UNCERTAINTY_ASSIGNED_CONTEXT((#14069))
GLOBAL_UNIT_ASSIGNED_CONTEXT((#14085,#14087,#14088))
REPRESENTATION_CONTEXT('','3D')
);
#14084=(
GEOMETRIC_REPRESENTATION_CONTEXT(3)
GLOBAL_UNCERTAINTY_ASSIGNED_CONTEXT((#14073))
GLOBAL_UNIT_ASSIGNED_CONTEXT((#14085,#14087,#14088))
REPRESENTATION_CONTEXT('','3D')
);
#14085=(
LENGTH_UNIT()
NAMED_UNIT(*)
SI_UNIT(.MILLI.,.METRE.)
);
#14087=(
NAMED_UNIT(*)
PLANE_ANGLE_UNIT()
SI_UNIT($,.RADIAN.)
);
#14088=(
NAMED_UNIT(*)
SI_UNIT($,.STERADIAN.)
SOLID_ANGLE_UNIT()
);
#14095=SHAPE_DEFINITION_REPRESENTATION(#14105,#14125);
#14105=PRODUCT_DEFINITION_SHAPE('',$,#14136);
#14125=SHAPE_REPRESENTATION('',(#3763),#14080);
#14129=PRODUCT_DEFINITION_CONTEXT('part definition',#14161,'design');
#14136=PRODUCT_DEFINITION('trigger','trigger',#14146,#14129);
#14146=PRODUCT_DEFINITION_FORMATION('',$,#14169);
#14161=APPLICATION_CONTEXT(
'Core Data for Automotive Mechanical Design Process');
#14162=PRODUCT_CONTEXT('part definition',#14161,'mechanical');
#14169=PRODUCT('trigger','trigger',$,(#14162));
#14175=PRESENTATION_STYLE_ASSIGNMENT((#14181));
#14181=SURFACE_STYLE_USAGE(.BOTH.,#14187);
#14187=SURFACE_SIDE_STYLE('',(#14193));
#14193=SURFACE_STYLE_FILL_AREA(#14199);
#14199=FILL_AREA_STYLE('Opaque(227,224,212)',(#14205));
#14205=FILL_AREA_STYLE_COLOUR('Opaque(227,224,212)',#14211);
#14211=COLOUR_RGB('Opaque(227,224,212)',0.890196078431372,0.87843137254902,
0.831372549019608);
ENDSEC;
END-ISO-10303-21;
